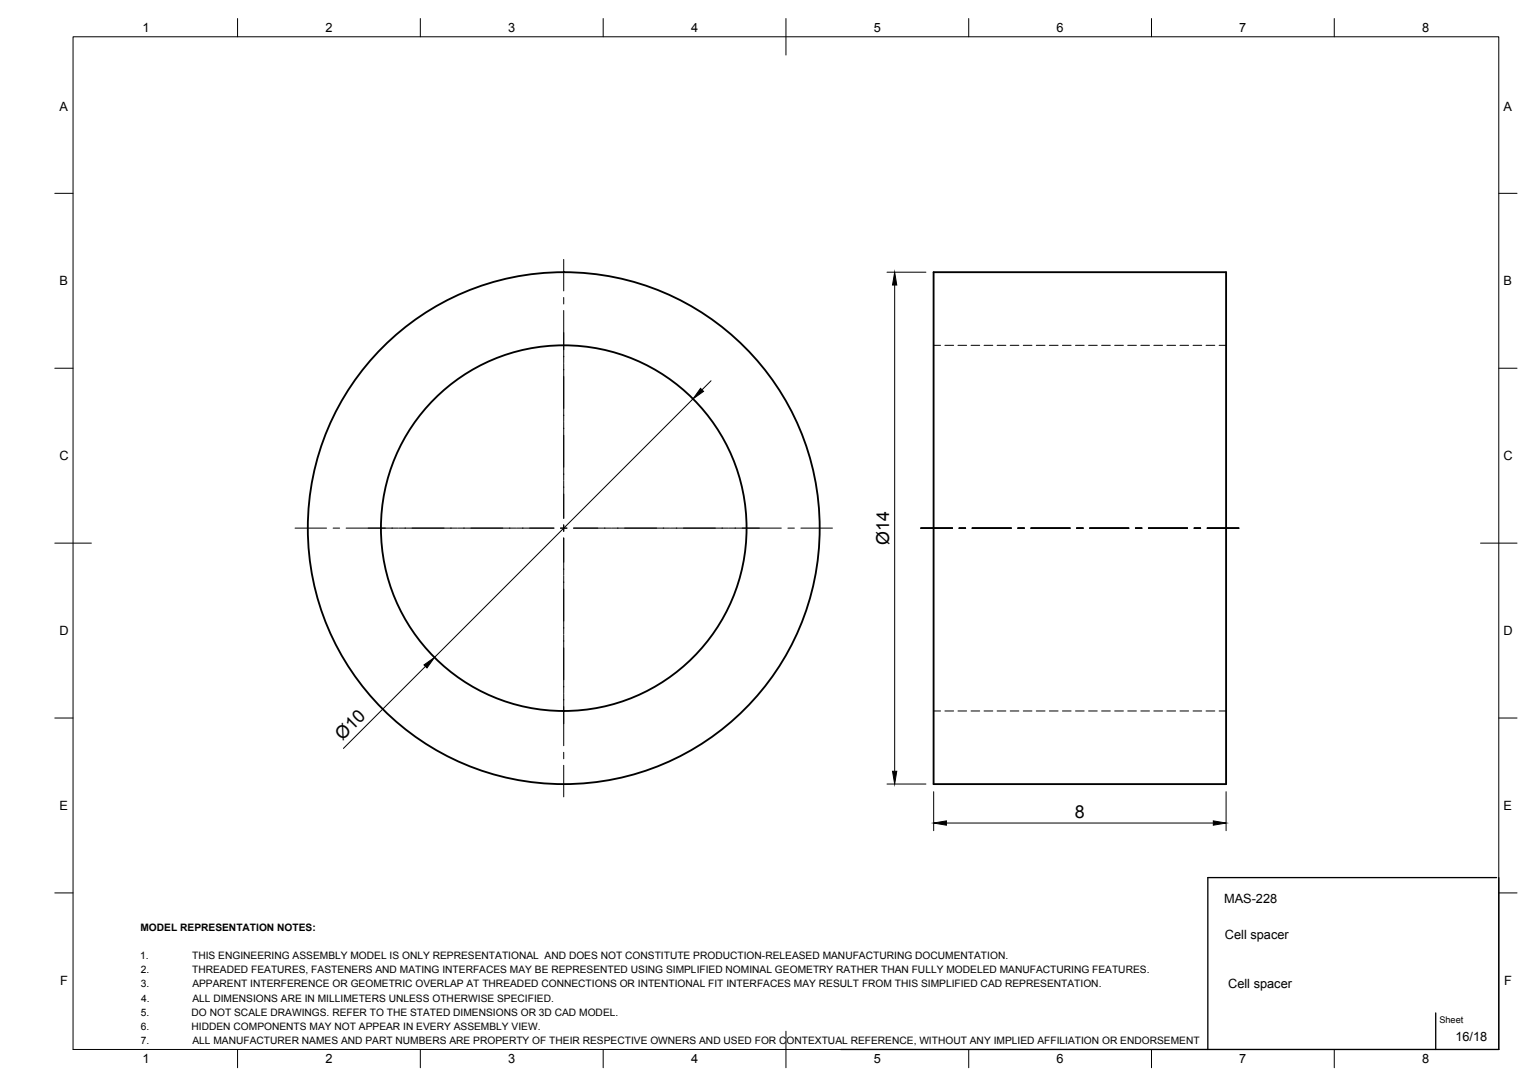
ISO-10303-21;
HEADER;
/* Generated by software containing ST-Developer
 * from STEP Tools, Inc. (www.steptools.com) 
 */

FILE_DESCRIPTION(
/* description */ ('Independent Peaucellier-Lipkin straight-line linkage. Radius arms 100
 mm, inversion-cell links 60 mm, crank radius and fixed-pivot spacing 
32 mm. Inversion constant 6400 mm squared, nominal output straight lin
e X=100 mm. Overhead bearing bridge clears the layered moving links. N
o accuracy or load rating assigned.'),
/* implementation_level */ '2;1');

FILE_NAME(
/* name */ 'Cell spacer.step',
/* time_stamp */ '2026-11-09T18:06:16-08:00',
/* author */ (''),
/* organization */ (''),
/* preprocessor_version */ 'ST-DEVELOPER v20.2',
/* originating_system */ 'Autodesk Translation Framework v15.17.0.0',
/* authorisation */ '');

FILE_SCHEMA (('AUTOMOTIVE_DESIGN { 1 0 10303 214 3 1 1 }'));
ENDSEC;

DATA;
#10=MECHANICAL_DESIGN_GEOMETRIC_PRESENTATION_REPRESENTATION('',(#296),#3581);
#262=SHAPE_REPRESENTATION_RELATIONSHIP('SRR','None',#3696,#279);
#279=ADVANCED_BREP_SHAPE_REPRESENTATION('',(#313),#3578);
#296=STYLED_ITEM('',(#3783),#313);
#313=MANIFOLD_SOLID_BREP('Body1',#1882);
#360=FACE_BOUND('',#680,.T.);
#361=FACE_BOUND('',#682,.T.);
#417=PLANE('',#2278);
#418=PLANE('',#2279);
#522=FACE_OUTER_BOUND('',#677,.T.);
#523=FACE_OUTER_BOUND('',#678,.T.);
#524=FACE_OUTER_BOUND('',#679,.T.);
#525=FACE_OUTER_BOUND('',#681,.T.);
#677=EDGE_LOOP('',(#1660,#1661,#1662,#1663));
#678=EDGE_LOOP('',(#1664,#1665,#1666,#1667));
#679=EDGE_LOOP('',(#1668));
#680=EDGE_LOOP('',(#1669));
#681=EDGE_LOOP('',(#1670));
#682=EDGE_LOOP('',(#1671));
#781=LINE('',#3433,#879);
#782=LINE('',#3439,#880);
#879=VECTOR('',#2847,5.);
#880=VECTOR('',#2854,7.);
#977=CIRCLE('',#2273,5.);
#978=CIRCLE('',#2274,5.);
#979=CIRCLE('',#2276,7.);
#980=CIRCLE('',#2277,7.);
#1104=VERTEX_POINT('',#3430);
#1105=VERTEX_POINT('',#3432);
#1106=VERTEX_POINT('',#3436);
#1107=VERTEX_POINT('',#3438);
#1292=EDGE_CURVE('',#1104,#1104,#977,.T.);
#1293=EDGE_CURVE('',#1104,#1105,#781,.T.);
#1294=EDGE_CURVE('',#1105,#1105,#978,.T.);
#1295=EDGE_CURVE('',#1106,#1106,#979,.T.);
#1296=EDGE_CURVE('',#1106,#1107,#782,.T.);
#1297=EDGE_CURVE('',#1107,#1107,#980,.T.);
#1660=ORIENTED_EDGE('',*,*,#1292,.F.);
#1661=ORIENTED_EDGE('',*,*,#1293,.T.);
#1662=ORIENTED_EDGE('',*,*,#1294,.T.);
#1663=ORIENTED_EDGE('',*,*,#1293,.F.);
#1664=ORIENTED_EDGE('',*,*,#1295,.F.);
#1665=ORIENTED_EDGE('',*,*,#1296,.T.);
#1666=ORIENTED_EDGE('',*,*,#1297,.T.);
#1667=ORIENTED_EDGE('',*,*,#1296,.F.);
#1668=ORIENTED_EDGE('',*,*,#1295,.T.);
#1669=ORIENTED_EDGE('',*,*,#1292,.T.);
#1670=ORIENTED_EDGE('',*,*,#1297,.F.);
#1671=ORIENTED_EDGE('',*,*,#1294,.F.);
#1751=CYLINDRICAL_SURFACE('',#2272,5.);
#1752=CYLINDRICAL_SURFACE('',#2275,7.);
#1854=ADVANCED_FACE('',(#522),#1751,.F.);
#1855=ADVANCED_FACE('',(#523),#1752,.T.);
#1856=ADVANCED_FACE('',(#524,#360),#417,.T.);
#1857=ADVANCED_FACE('',(#525,#361),#418,.F.);
#1882=CLOSED_SHELL('',(#1854,#1855,#1856,#1857));
#2271=AXIS2_PLACEMENT_3D('',#3428,#2841,#2842);
#2272=AXIS2_PLACEMENT_3D('',#3429,#2843,#2844);
#2273=AXIS2_PLACEMENT_3D('',#3431,#2845,#2846);
#2274=AXIS2_PLACEMENT_3D('',#3434,#2848,#2849);
#2275=AXIS2_PLACEMENT_3D('',#3435,#2850,#2851);
#2276=AXIS2_PLACEMENT_3D('',#3437,#2852,#2853);
#2277=AXIS2_PLACEMENT_3D('',#3440,#2855,#2856);
#2278=AXIS2_PLACEMENT_3D('',#3441,#2857,#2858);
#2279=AXIS2_PLACEMENT_3D('',#3442,#2859,#2860);
#2841=DIRECTION('axis',(0.,0.,1.));
#2842=DIRECTION('refdir',(1.,0.,0.));
#2843=DIRECTION('center_axis',(0.,0.,1.));
#2844=DIRECTION('ref_axis',(1.,0.,0.));
#2845=DIRECTION('center_axis',(0.,0.,-1.));
#2846=DIRECTION('ref_axis',(1.,0.,0.));
#2847=DIRECTION('',(0.,0.,-1.));
#2848=DIRECTION('center_axis',(0.,0.,-1.));
#2849=DIRECTION('ref_axis',(1.,0.,0.));
#2850=DIRECTION('center_axis',(0.,0.,1.));
#2851=DIRECTION('ref_axis',(1.,0.,0.));
#2852=DIRECTION('center_axis',(0.,0.,1.));
#2853=DIRECTION('ref_axis',(1.,0.,0.));
#2854=DIRECTION('',(0.,0.,-1.));
#2855=DIRECTION('center_axis',(0.,0.,1.));
#2856=DIRECTION('ref_axis',(1.,0.,0.));
#2857=DIRECTION('center_axis',(0.,0.,1.));
#2858=DIRECTION('ref_axis',(1.,0.,0.));
#2859=DIRECTION('center_axis',(0.,0.,1.));
#2860=DIRECTION('ref_axis',(1.,0.,0.));
#3428=CARTESIAN_POINT('',(0.,0.,0.));
#3429=CARTESIAN_POINT('Origin',(0.,0.,0.));
#3430=CARTESIAN_POINT('',(-5.,-6.12323399573677E-16,8.));
#3431=CARTESIAN_POINT('Origin',(0.,0.,8.));
#3432=CARTESIAN_POINT('',(-5.,-6.12323399573677E-16,0.));
#3433=CARTESIAN_POINT('',(-5.,-6.12323399573677E-16,0.));
#3434=CARTESIAN_POINT('Origin',(0.,0.,0.));
#3435=CARTESIAN_POINT('Origin',(0.,0.,0.));
#3436=CARTESIAN_POINT('',(-7.,-8.57252759403147E-16,8.));
#3437=CARTESIAN_POINT('Origin',(0.,0.,8.));
#3438=CARTESIAN_POINT('',(-7.,-8.57252759403147E-16,0.));
#3439=CARTESIAN_POINT('',(-7.,-8.57252759403147E-16,0.));
#3440=CARTESIAN_POINT('Origin',(0.,0.,0.));
#3441=CARTESIAN_POINT('Origin',(0.,0.,8.));
#3442=CARTESIAN_POINT('Origin',(0.,0.,0.));
#3559=UNCERTAINTY_MEASURE_WITH_UNIT(LENGTH_MEASURE(0.01),#3582,
'DISTANCE_ACCURACY_VALUE',
'Maximum model space distance between geometric entities at asserted c
onnectivities');
#3562=UNCERTAINTY_MEASURE_WITH_UNIT(LENGTH_MEASURE(0.01),#3582,
'DISTANCE_ACCURACY_VALUE',
'Maximum model space distance between geometric entities at asserted c
onnectivities');
#3578=(
GEOMETRIC_REPRESENTATION_CONTEXT(3)
GLOBAL_UNCERTAINTY_ASSIGNED_CONTEXT((#3559))
GLOBAL_UNIT_ASSIGNED_CONTEXT((#3582,#3584,#3585))
REPRESENTATION_CONTEXT('','3D')
);
#3581=(
GEOMETRIC_REPRESENTATION_CONTEXT(3)
GLOBAL_UNCERTAINTY_ASSIGNED_CONTEXT((#3562))
GLOBAL_UNIT_ASSIGNED_CONTEXT((#3582,#3584,#3585))
REPRESENTATION_CONTEXT('','3D')
);
#3582=(
LENGTH_UNIT()
NAMED_UNIT(*)
SI_UNIT(.MILLI.,.METRE.)
);
#3584=(
NAMED_UNIT(*)
PLANE_ANGLE_UNIT()
SI_UNIT($,.RADIAN.)
);
#3585=(
NAMED_UNIT(*)
SI_UNIT($,.STERADIAN.)
SOLID_ANGLE_UNIT()
);
#3601=SHAPE_DEFINITION_REPRESENTATION(#3619,#3696);
#3619=PRODUCT_DEFINITION_SHAPE('',$,#3715);
#3696=SHAPE_REPRESENTATION('',(#2271),#3578);
#3699=PRODUCT_DEFINITION_CONTEXT('part definition',#3755,'design');
#3715=PRODUCT_DEFINITION('Cell spacer','Cell spacer',#3733,#3699);
#3733=PRODUCT_DEFINITION_FORMATION('',$,#3772);
#3755=APPLICATION_CONTEXT(
'Core Data for Automotive Mechanical Design Process');
#3756=PRODUCT_CONTEXT('part definition',#3755,'mechanical');
#3772=PRODUCT('Cell spacer','Cell spacer',$,(#3756));
#3783=PRESENTATION_STYLE_ASSIGNMENT((#3796));
#3796=SURFACE_STYLE_USAGE(.BOTH.,#3809);
#3809=SURFACE_SIDE_STYLE('',(#3822));
#3822=SURFACE_STYLE_FILL_AREA(#3835);
#3835=FILL_AREA_STYLE('Spacer light gray',(#3848));
#3848=FILL_AREA_STYLE_COLOUR('Spacer light gray',#3861);
#3861=COLOUR_RGB('Spacer light gray',0.725490196078431,0.752941176470588,
0.792156862745098);
ENDSEC;
END-ISO-10303-21;
